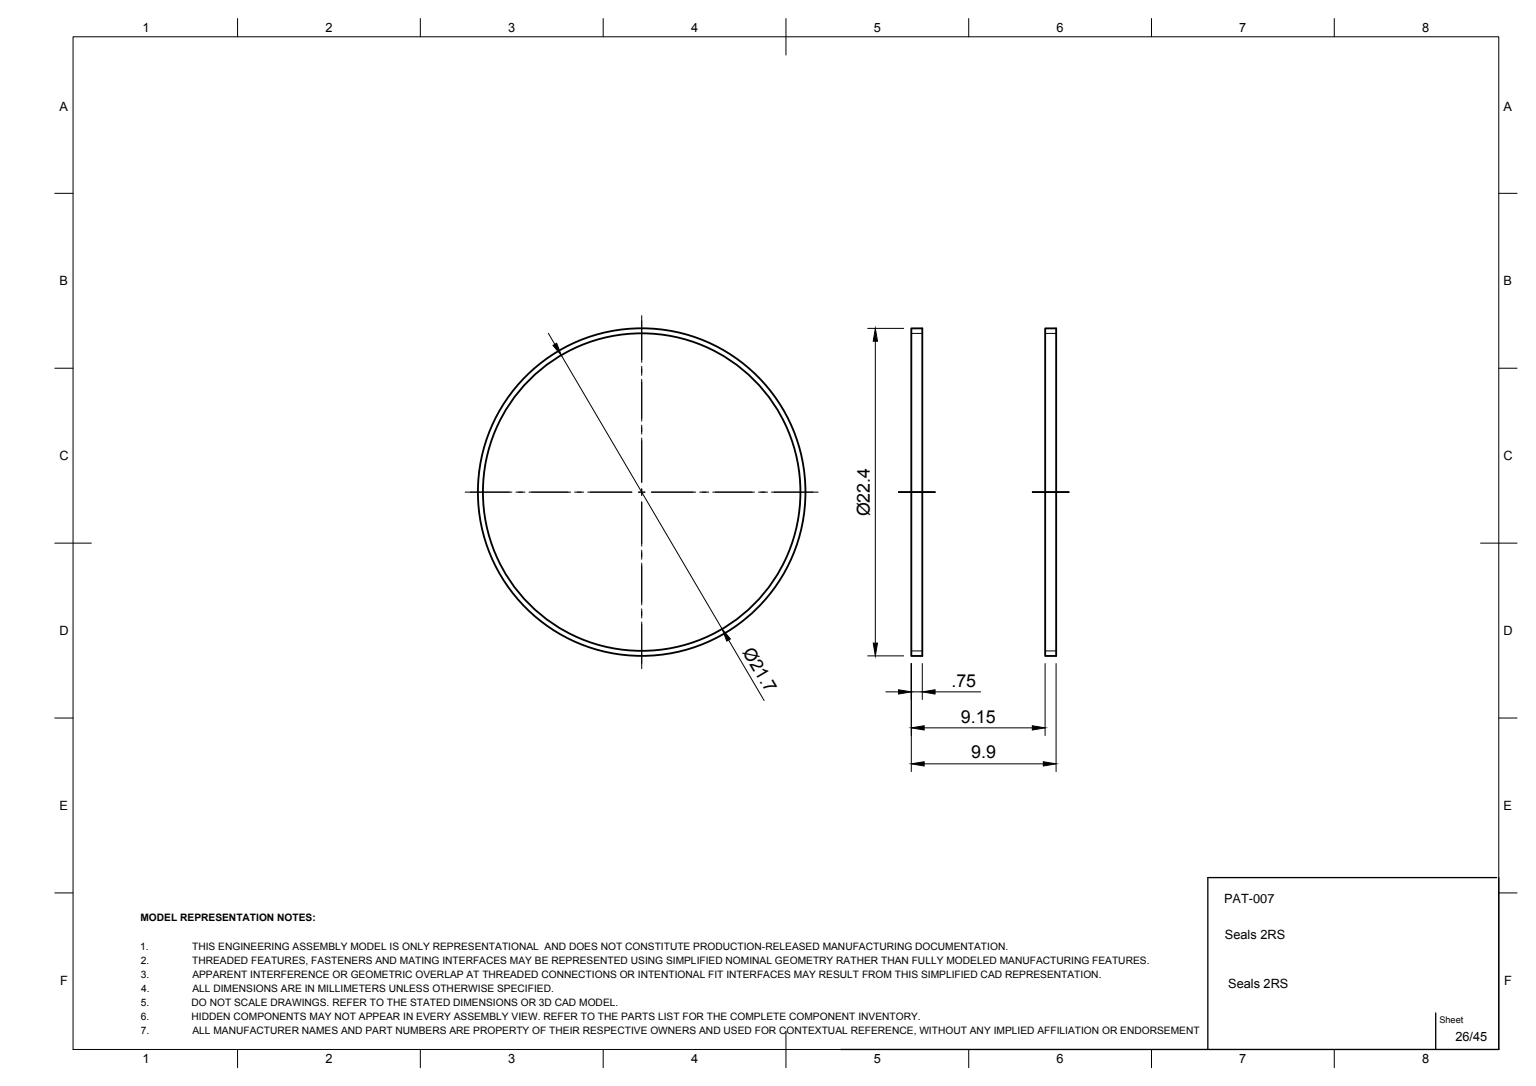
ISO-10303-21;
HEADER;
/* Generated by software containing ST-Developer
 * from STEP Tools, Inc. (www.steptools.com) 
 */

FILE_DESCRIPTION(
/* description */ ('Bearing friction torque test rig'),
/* implementation_level */ '2;1');

FILE_NAME(
/* name */ 'Seals 2RS.step',
/* time_stamp */ '2026-10-28T03:24:04-07:00',
/* author */ (''),
/* organization */ (''),
/* preprocessor_version */ 'ST-DEVELOPER v20.2',
/* originating_system */ 'Autodesk Translation Framework v15.17.0.0',
/* authorisation */ '');

FILE_SCHEMA (('AUTOMOTIVE_DESIGN { 1 0 10303 214 3 1 1 }'));
ENDSEC;

DATA;
#10=MECHANICAL_DESIGN_GEOMETRIC_PRESENTATION_REPRESENTATION('',(#565,#566),#14822);
#481=SHAPE_REPRESENTATION_RELATIONSHIP('SRR','None',#15021,#520);
#520=ADVANCED_BREP_SHAPE_REPRESENTATION('',(#618,#619),#14801);
#565=STYLED_ITEM('',(#15284),#618);
#566=STYLED_ITEM('',(#15284),#619);
#618=MANIFOLD_SOLID_BREP('Body1',#7682);
#619=MANIFOLD_SOLID_BREP('Body2',#7683);
#819=FACE_BOUND('',#1997,.T.);
#820=FACE_BOUND('',#2000,.T.);
#821=FACE_BOUND('',#2003,.T.);
#822=FACE_BOUND('',#2006,.T.);
#1014=PLANE('',#8729);
#1015=PLANE('',#8734);
#1016=PLANE('',#8737);
#1017=PLANE('',#8742);
#1376=FACE_OUTER_BOUND('',#1996,.T.);
#1377=FACE_OUTER_BOUND('',#1998,.T.);
#1378=FACE_OUTER_BOUND('',#1999,.T.);
#1379=FACE_OUTER_BOUND('',#2001,.T.);
#1380=FACE_OUTER_BOUND('',#2002,.T.);
#1381=FACE_OUTER_BOUND('',#2004,.T.);
#1382=FACE_OUTER_BOUND('',#2005,.T.);
#1383=FACE_OUTER_BOUND('',#2007,.T.);
#1996=EDGE_LOOP('',(#6378));
#1997=EDGE_LOOP('',(#6379));
#1998=EDGE_LOOP('',(#6380,#6381,#6382,#6383));
#1999=EDGE_LOOP('',(#6384));
#2000=EDGE_LOOP('',(#6385));
#2001=EDGE_LOOP('',(#6386,#6387,#6388,#6389));
#2002=EDGE_LOOP('',(#6390));
#2003=EDGE_LOOP('',(#6391));
#2004=EDGE_LOOP('',(#6392,#6393,#6394,#6395));
#2005=EDGE_LOOP('',(#6396));
#2006=EDGE_LOOP('',(#6397));
#2007=EDGE_LOOP('',(#6398,#6399,#6400,#6401));
#2534=LINE('',#13293,#2978);
#2535=LINE('',#13298,#2979);
#2536=LINE('',#13307,#2980);
#2537=LINE('',#13312,#2981);
#2978=VECTOR('',#10665,1.119765);
#2979=VECTOR('',#10672,1.085235);
#2980=VECTOR('',#10683,1.119765);
#2981=VECTOR('',#10690,1.085235);
#3387=CIRCLE('',#8730,1.119765);
#3388=CIRCLE('',#8731,1.085235);
#3389=CIRCLE('',#8733,1.119765);
#3390=CIRCLE('',#8735,1.085235);
#3391=CIRCLE('',#8738,1.119765);
#3392=CIRCLE('',#8739,1.085235);
#3393=CIRCLE('',#8741,1.119765);
#3394=CIRCLE('',#8743,1.085235);
#3970=VERTEX_POINT('',#13286);
#3971=VERTEX_POINT('',#13288);
#3972=VERTEX_POINT('',#13291);
#3973=VERTEX_POINT('',#13295);
#3974=VERTEX_POINT('',#13300);
#3975=VERTEX_POINT('',#13302);
#3976=VERTEX_POINT('',#13305);
#3977=VERTEX_POINT('',#13309);
#4815=EDGE_CURVE('',#3970,#3970,#3387,.T.);
#4816=EDGE_CURVE('',#3971,#3971,#3388,.T.);
#4817=EDGE_CURVE('',#3972,#3972,#3389,.T.);
#4818=EDGE_CURVE('',#3972,#3970,#2534,.T.);
#4819=EDGE_CURVE('',#3973,#3973,#3390,.T.);
#4820=EDGE_CURVE('',#3973,#3971,#2535,.T.);
#4821=EDGE_CURVE('',#3974,#3974,#3391,.T.);
#4822=EDGE_CURVE('',#3975,#3975,#3392,.T.);
#4823=EDGE_CURVE('',#3976,#3976,#3393,.T.);
#4824=EDGE_CURVE('',#3976,#3974,#2536,.T.);
#4825=EDGE_CURVE('',#3977,#3977,#3394,.T.);
#4826=EDGE_CURVE('',#3977,#3975,#2537,.T.);
#6378=ORIENTED_EDGE('',*,*,#4815,.F.);
#6379=ORIENTED_EDGE('',*,*,#4816,.T.);
#6380=ORIENTED_EDGE('',*,*,#4817,.F.);
#6381=ORIENTED_EDGE('',*,*,#4818,.T.);
#6382=ORIENTED_EDGE('',*,*,#4815,.T.);
#6383=ORIENTED_EDGE('',*,*,#4818,.F.);
#6384=ORIENTED_EDGE('',*,*,#4817,.T.);
#6385=ORIENTED_EDGE('',*,*,#4819,.F.);
#6386=ORIENTED_EDGE('',*,*,#4819,.T.);
#6387=ORIENTED_EDGE('',*,*,#4820,.T.);
#6388=ORIENTED_EDGE('',*,*,#4816,.F.);
#6389=ORIENTED_EDGE('',*,*,#4820,.F.);
#6390=ORIENTED_EDGE('',*,*,#4821,.F.);
#6391=ORIENTED_EDGE('',*,*,#4822,.T.);
#6392=ORIENTED_EDGE('',*,*,#4823,.F.);
#6393=ORIENTED_EDGE('',*,*,#4824,.T.);
#6394=ORIENTED_EDGE('',*,*,#4821,.T.);
#6395=ORIENTED_EDGE('',*,*,#4824,.F.);
#6396=ORIENTED_EDGE('',*,*,#4823,.T.);
#6397=ORIENTED_EDGE('',*,*,#4825,.F.);
#6398=ORIENTED_EDGE('',*,*,#4825,.T.);
#6399=ORIENTED_EDGE('',*,*,#4826,.T.);
#6400=ORIENTED_EDGE('',*,*,#4822,.F.);
#6401=ORIENTED_EDGE('',*,*,#4826,.F.);
#7158=CYLINDRICAL_SURFACE('',#8732,1.119765);
#7159=CYLINDRICAL_SURFACE('',#8736,1.085235);
#7160=CYLINDRICAL_SURFACE('',#8740,1.119765);
#7161=CYLINDRICAL_SURFACE('',#8744,1.085235);
#7487=ADVANCED_FACE('',(#1376,#819),#1014,.T.);
#7488=ADVANCED_FACE('',(#1377),#7158,.T.);
#7489=ADVANCED_FACE('',(#1378,#820),#1015,.T.);
#7490=ADVANCED_FACE('',(#1379),#7159,.F.);
#7491=ADVANCED_FACE('',(#1380,#821),#1016,.T.);
#7492=ADVANCED_FACE('',(#1381),#7160,.T.);
#7493=ADVANCED_FACE('',(#1382,#822),#1017,.T.);
#7494=ADVANCED_FACE('',(#1383),#7161,.F.);
#7682=CLOSED_SHELL('',(#7487,#7488,#7489,#7490));
#7683=CLOSED_SHELL('',(#7491,#7492,#7493,#7494));
#8728=AXIS2_PLACEMENT_3D('',#13284,#10653,#10654);
#8729=AXIS2_PLACEMENT_3D('',#13285,#10655,#10656);
#8730=AXIS2_PLACEMENT_3D('',#13287,#10657,#10658);
#8731=AXIS2_PLACEMENT_3D('',#13289,#10659,#10660);
#8732=AXIS2_PLACEMENT_3D('',#13290,#10661,#10662);
#8733=AXIS2_PLACEMENT_3D('',#13292,#10663,#10664);
#8734=AXIS2_PLACEMENT_3D('',#13294,#10666,#10667);
#8735=AXIS2_PLACEMENT_3D('',#13296,#10668,#10669);
#8736=AXIS2_PLACEMENT_3D('',#13297,#10670,#10671);
#8737=AXIS2_PLACEMENT_3D('',#13299,#10673,#10674);
#8738=AXIS2_PLACEMENT_3D('',#13301,#10675,#10676);
#8739=AXIS2_PLACEMENT_3D('',#13303,#10677,#10678);
#8740=AXIS2_PLACEMENT_3D('',#13304,#10679,#10680);
#8741=AXIS2_PLACEMENT_3D('',#13306,#10681,#10682);
#8742=AXIS2_PLACEMENT_3D('',#13308,#10684,#10685);
#8743=AXIS2_PLACEMENT_3D('',#13310,#10686,#10687);
#8744=AXIS2_PLACEMENT_3D('',#13311,#10688,#10689);
#10653=DIRECTION('axis',(0.,0.,1.));
#10654=DIRECTION('refdir',(1.,0.,0.));
#10655=DIRECTION('center_axis',(0.,1.,0.));
#10656=DIRECTION('ref_axis',(0.,0.,1.));
#10657=DIRECTION('center_axis',(0.,-1.,0.));
#10658=DIRECTION('ref_axis',(1.,0.,0.));
#10659=DIRECTION('center_axis',(0.,-1.,0.));
#10660=DIRECTION('ref_axis',(1.,0.,0.));
#10661=DIRECTION('center_axis',(0.,-1.,0.));
#10662=DIRECTION('ref_axis',(1.,0.,0.));
#10663=DIRECTION('center_axis',(0.,-1.,0.));
#10664=DIRECTION('ref_axis',(1.,0.,0.));
#10665=DIRECTION('',(0.,1.,0.));
#10666=DIRECTION('center_axis',(0.,-1.,0.));
#10667=DIRECTION('ref_axis',(0.,0.,-1.));
#10668=DIRECTION('center_axis',(0.,-1.,0.));
#10669=DIRECTION('ref_axis',(1.,0.,0.));
#10670=DIRECTION('center_axis',(0.,-1.,0.));
#10671=DIRECTION('ref_axis',(1.,0.,0.));
#10672=DIRECTION('',(0.,1.,0.));
#10673=DIRECTION('center_axis',(0.,1.,0.));
#10674=DIRECTION('ref_axis',(0.,0.,1.));
#10675=DIRECTION('center_axis',(0.,-1.,0.));
#10676=DIRECTION('ref_axis',(1.,0.,0.));
#10677=DIRECTION('center_axis',(0.,-1.,0.));
#10678=DIRECTION('ref_axis',(1.,0.,0.));
#10679=DIRECTION('center_axis',(0.,-1.,0.));
#10680=DIRECTION('ref_axis',(1.,0.,0.));
#10681=DIRECTION('center_axis',(0.,-1.,0.));
#10682=DIRECTION('ref_axis',(1.,0.,0.));
#10683=DIRECTION('',(0.,1.,0.));
#10684=DIRECTION('center_axis',(0.,-1.,0.));
#10685=DIRECTION('ref_axis',(0.,0.,-1.));
#10686=DIRECTION('center_axis',(0.,-1.,0.));
#10687=DIRECTION('ref_axis',(1.,0.,0.));
#10688=DIRECTION('center_axis',(0.,-1.,0.));
#10689=DIRECTION('ref_axis',(1.,0.,0.));
#10690=DIRECTION('',(0.,1.,0.));
#13284=CARTESIAN_POINT('',(0.,0.,0.));
#13285=CARTESIAN_POINT('Origin',(1.119765,0.495,0.));
#13286=CARTESIAN_POINT('',(-1.119765,0.495,-1.37131662304724E-16));
#13287=CARTESIAN_POINT('Origin',(0.,0.495,0.));
#13288=CARTESIAN_POINT('',(-1.085235,0.495,-1.32902956907268E-16));
#13289=CARTESIAN_POINT('Origin',(0.,0.495,0.));
#13290=CARTESIAN_POINT('Origin',(0.,0.4575,0.));
#13291=CARTESIAN_POINT('',(-1.119765,0.42,-1.37131662304724E-16));
#13292=CARTESIAN_POINT('Origin',(0.,0.42,0.));
#13293=CARTESIAN_POINT('',(-1.119765,0.4575,-1.37131662304724E-16));
#13294=CARTESIAN_POINT('Origin',(1.085235,0.42,0.));
#13295=CARTESIAN_POINT('',(-1.085235,0.42,-1.32902956907268E-16));
#13296=CARTESIAN_POINT('Origin',(0.,0.42,0.));
#13297=CARTESIAN_POINT('Origin',(0.,0.4575,0.));
#13298=CARTESIAN_POINT('',(-1.085235,0.4575,-1.32902956907268E-16));
#13299=CARTESIAN_POINT('Origin',(1.119765,-0.42,0.));
#13300=CARTESIAN_POINT('',(-1.119765,-0.42,-1.37131662304724E-16));
#13301=CARTESIAN_POINT('Origin',(0.,-0.42,0.));
#13302=CARTESIAN_POINT('',(-1.085235,-0.42,-1.32902956907268E-16));
#13303=CARTESIAN_POINT('Origin',(0.,-0.42,0.));
#13304=CARTESIAN_POINT('Origin',(0.,-0.4575,0.));
#13305=CARTESIAN_POINT('',(-1.119765,-0.495,-1.37131662304724E-16));
#13306=CARTESIAN_POINT('Origin',(0.,-0.495,0.));
#13307=CARTESIAN_POINT('',(-1.119765,-0.4575,-1.37131662304724E-16));
#13308=CARTESIAN_POINT('Origin',(1.085235,-0.495,0.));
#13309=CARTESIAN_POINT('',(-1.085235,-0.495,-1.32902956907268E-16));
#13310=CARTESIAN_POINT('Origin',(0.,-0.495,0.));
#13311=CARTESIAN_POINT('Origin',(0.,-0.4575,0.));
#13312=CARTESIAN_POINT('',(-1.085235,-0.4575,-1.32902956907268E-16));
#14756=UNCERTAINTY_MEASURE_WITH_UNIT(LENGTH_MEASURE(0.001),#14823,
'DISTANCE_ACCURACY_VALUE',
'Maximum model space distance between geometric entities at asserted c
onnectivities');
#14777=UNCERTAINTY_MEASURE_WITH_UNIT(LENGTH_MEASURE(0.001),#14823,
'DISTANCE_ACCURACY_VALUE',
'Maximum model space distance between geometric entities at asserted c
onnectivities');
#14801=(
GEOMETRIC_REPRESENTATION_CONTEXT(3)
GLOBAL_UNCERTAINTY_ASSIGNED_CONTEXT((#14756))
GLOBAL_UNIT_ASSIGNED_CONTEXT((#14823,#14825,#14826))
REPRESENTATION_CONTEXT('','3D')
);
#14822=(
GEOMETRIC_REPRESENTATION_CONTEXT(3)
GLOBAL_UNCERTAINTY_ASSIGNED_CONTEXT((#14777))
GLOBAL_UNIT_ASSIGNED_CONTEXT((#14823,#14825,#14826))
REPRESENTATION_CONTEXT('','3D')
);
#14823=(
LENGTH_UNIT()
NAMED_UNIT(*)
SI_UNIT(.CENTI.,.METRE.)
);
#14825=(
NAMED_UNIT(*)
PLANE_ANGLE_UNIT()
SI_UNIT($,.RADIAN.)
);
#14826=(
NAMED_UNIT(*)
SI_UNIT($,.STERADIAN.)
SOLID_ANGLE_UNIT()
);
#14850=SHAPE_DEFINITION_REPRESENTATION(#14894,#15021);
#14894=PRODUCT_DEFINITION_SHAPE('',$,#15066);
#15021=SHAPE_REPRESENTATION('',(#8728),#14801);
#15042=PRODUCT_DEFINITION_CONTEXT('part definition',#15176,'design');
#15066=PRODUCT_DEFINITION('Seals 2RS','Seals 2RS',#15110,#15042);
#15110=PRODUCT_DEFINITION_FORMATION('',$,#15201);
#15176=APPLICATION_CONTEXT(
'Core Data for Automotive Mechanical Design Process');
#15177=PRODUCT_CONTEXT('part definition',#15176,'mechanical');
#15201=PRODUCT('Seals 2RS','Seals 2RS','Seals 2RS',(#15177));
#15278=COLOUR_RGB('Grey',0.48,0.52,0.57);
#15279=FILL_AREA_STYLE_COLOUR('',#15278);
#15280=FILL_AREA_STYLE('',(#15279));
#15281=SURFACE_STYLE_FILL_AREA(#15280);
#15282=SURFACE_SIDE_STYLE('',(#15281));
#15283=SURFACE_STYLE_USAGE(.BOTH.,#15282);
#15284=PRESENTATION_STYLE_ASSIGNMENT((#15283));
ENDSEC;
END-ISO-10303-21;
